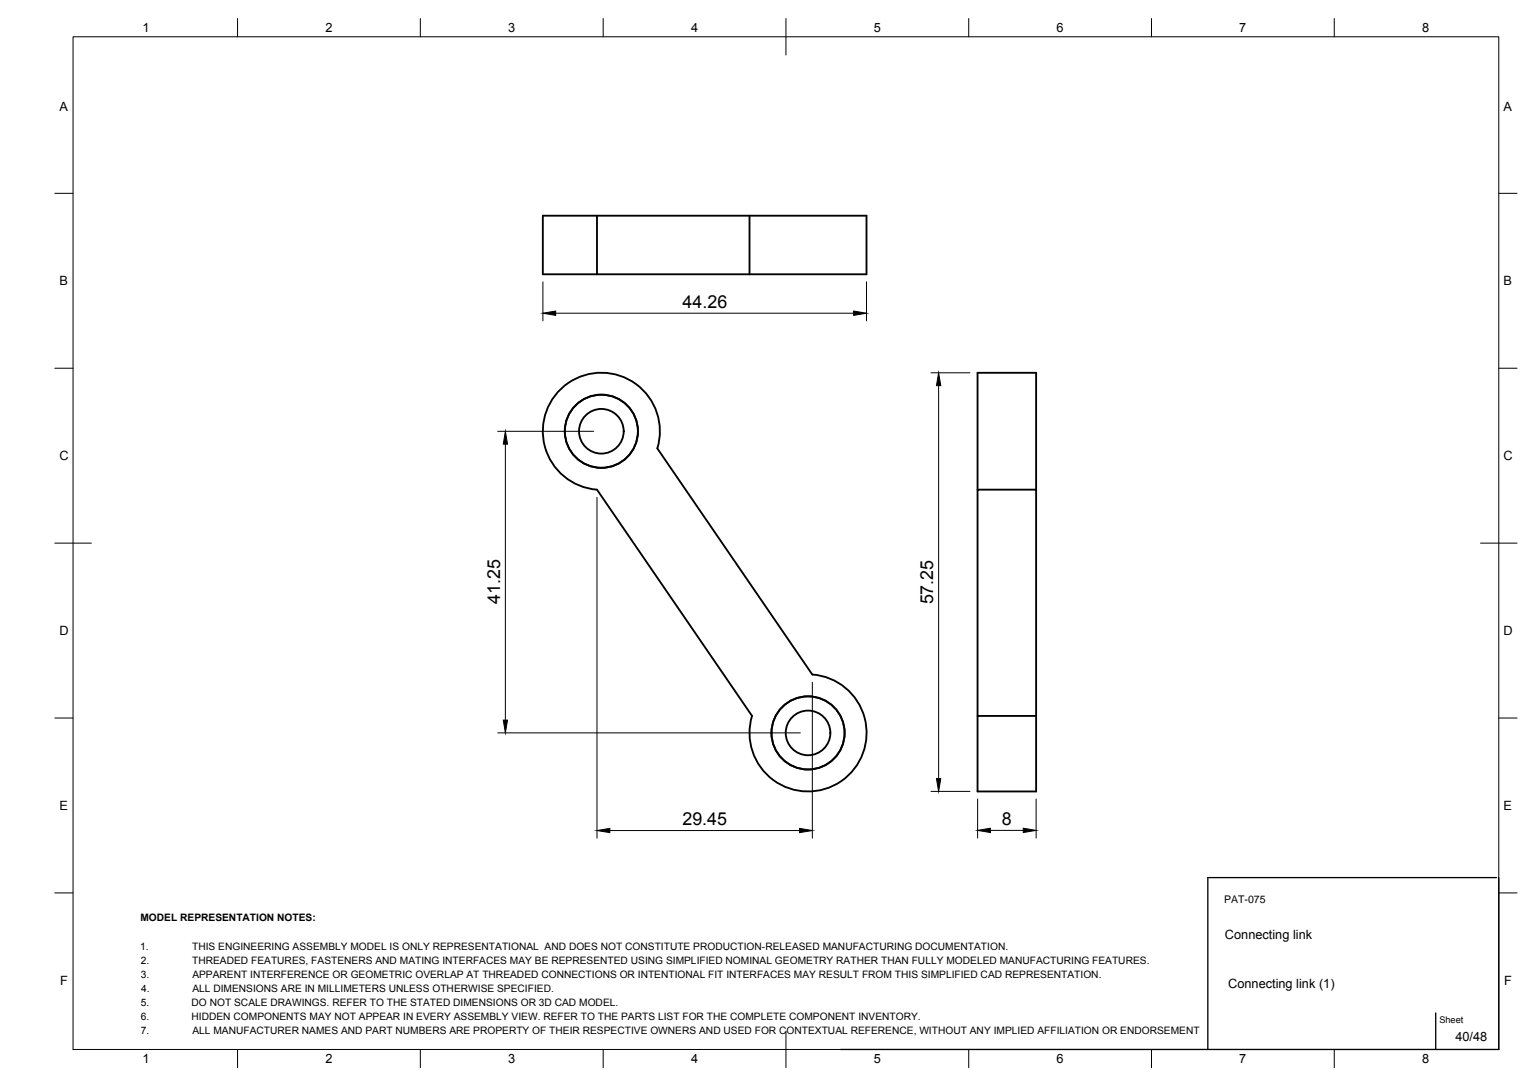
ISO-10303-21;
HEADER;
/* Generated by software containing ST-Developer
 * from STEP Tools, Inc. (www.steptools.com) 
 */

FILE_DESCRIPTION(
/* description */ ('Over-Centre Plunger Toggle Clamp on Slotted Fixture Frame'),
/* implementation_level */ '2;1');

FILE_NAME(
/* name */ 
'Connecting link.step',
/* time_stamp */ '2026-10-28T03:23:24-07:00',
/* author */ (''),
/* organization */ (''),
/* preprocessor_version */ 'ST-DEVELOPER v20.2',
/* originating_system */ 'Autodesk Translation Framework v15.17.0.0',
/* authorisation */ '');

FILE_SCHEMA (('AUTOMOTIVE_DESIGN { 1 0 10303 214 3 1 1 }'));
ENDSEC;

DATA;
#10=MECHANICAL_DESIGN_GEOMETRIC_PRESENTATION_REPRESENTATION('',(#556),#15212);
#464=SHAPE_REPRESENTATION_RELATIONSHIP('SRR','None',#15442,#506);
#506=ADVANCED_BREP_SHAPE_REPRESENTATION('',(#603),#15204);
#556=STYLED_ITEM('',(#15712),#603);
#603=MANIFOLD_SOLID_BREP('Body1',#8292);
#768=FACE_BOUND('',#2161,.T.);
#769=FACE_BOUND('',#2162,.T.);
#770=FACE_BOUND('',#2166,.T.);
#771=FACE_BOUND('',#2167,.T.);
#1046=PLANE('',#9644);
#1047=PLANE('',#9645);
#1048=PLANE('',#9647);
#1049=PLANE('',#9650);
#1513=FACE_OUTER_BOUND('',#2156,.T.);
#1514=FACE_OUTER_BOUND('',#2157,.T.);
#1515=FACE_OUTER_BOUND('',#2158,.T.);
#1516=FACE_OUTER_BOUND('',#2159,.T.);
#1517=FACE_OUTER_BOUND('',#2160,.T.);
#1518=FACE_OUTER_BOUND('',#2163,.T.);
#1519=FACE_OUTER_BOUND('',#2164,.T.);
#1520=FACE_OUTER_BOUND('',#2165,.T.);
#2156=EDGE_LOOP('',(#7377,#7378,#7379,#7380));
#2157=EDGE_LOOP('',(#7381,#7382,#7383,#7384));
#2158=EDGE_LOOP('',(#7385,#7386,#7387,#7388));
#2159=EDGE_LOOP('',(#7389,#7390,#7391,#7392));
#2160=EDGE_LOOP('',(#7393,#7394,#7395,#7396));
#2161=EDGE_LOOP('',(#7397));
#2162=EDGE_LOOP('',(#7398));
#2163=EDGE_LOOP('',(#7399,#7400,#7401,#7402));
#2164=EDGE_LOOP('',(#7403,#7404,#7405,#7406));
#2165=EDGE_LOOP('',(#7407,#7408,#7409,#7410));
#2166=EDGE_LOOP('',(#7411));
#2167=EDGE_LOOP('',(#7412));
#2784=LINE('',#14822,#3414);
#2785=LINE('',#14828,#3415);
#2786=LINE('',#14833,#3416);
#2787=LINE('',#14837,#3417);
#2788=LINE('',#14841,#3418);
#2789=LINE('',#14843,#3419);
#2790=LINE('',#14844,#3420);
#2791=LINE('',#14847,#3421);
#2792=LINE('',#14851,#3422);
#2793=LINE('',#14852,#3423);
#3414=VECTOR('',#12055,0.5);
#3415=VECTOR('',#12062,0.5);
#3416=VECTOR('',#12067,1.);
#3417=VECTOR('',#12070,1.);
#3418=VECTOR('',#12075,1.);
#3419=VECTOR('',#12076,1.);
#3420=VECTOR('',#12077,1.);
#3421=VECTOR('',#12080,1.);
#3422=VECTOR('',#12085,1.);
#3423=VECTOR('',#12086,1.);
#3818=CIRCLE('',#9636,0.5);
#3819=CIRCLE('',#9637,0.5);
#3820=CIRCLE('',#9639,0.5);
#3821=CIRCLE('',#9640,0.5);
#3822=CIRCLE('',#9642,0.8);
#3823=CIRCLE('',#9643,0.8);
#3824=CIRCLE('',#9646,0.8);
#3825=CIRCLE('',#9649,0.8);
#4466=VERTEX_POINT('',#14819);
#4467=VERTEX_POINT('',#14821);
#4468=VERTEX_POINT('',#14825);
#4469=VERTEX_POINT('',#14827);
#4470=VERTEX_POINT('',#14831);
#4471=VERTEX_POINT('',#14832);
#4472=VERTEX_POINT('',#14834);
#4473=VERTEX_POINT('',#14836);
#4474=VERTEX_POINT('',#14840);
#4475=VERTEX_POINT('',#14842);
#4476=VERTEX_POINT('',#14846);
#4477=VERTEX_POINT('',#14850);
#5449=EDGE_CURVE('',#4466,#4466,#3818,.T.);
#5450=EDGE_CURVE('',#4466,#4467,#2784,.T.);
#5451=EDGE_CURVE('',#4467,#4467,#3819,.T.);
#5452=EDGE_CURVE('',#4468,#4468,#3820,.T.);
#5453=EDGE_CURVE('',#4468,#4469,#2785,.T.);
#5454=EDGE_CURVE('',#4469,#4469,#3821,.T.);
#5455=EDGE_CURVE('',#4470,#4471,#2786,.T.);
#5456=EDGE_CURVE('',#4472,#4470,#3822,.T.);
#5457=EDGE_CURVE('',#4473,#4472,#2787,.T.);
#5458=EDGE_CURVE('',#4473,#4471,#3823,.T.);
#5459=EDGE_CURVE('',#4471,#4474,#2788,.T.);
#5460=EDGE_CURVE('',#4475,#4474,#2789,.T.);
#5461=EDGE_CURVE('',#4470,#4475,#2790,.T.);
#5462=EDGE_CURVE('',#4476,#4473,#2791,.T.);
#5463=EDGE_CURVE('',#4474,#4476,#3824,.T.);
#5464=EDGE_CURVE('',#4477,#4472,#2792,.T.);
#5465=EDGE_CURVE('',#4476,#4477,#2793,.T.);
#5466=EDGE_CURVE('',#4475,#4477,#3825,.T.);
#7377=ORIENTED_EDGE('',*,*,#5449,.F.);
#7378=ORIENTED_EDGE('',*,*,#5450,.T.);
#7379=ORIENTED_EDGE('',*,*,#5451,.F.);
#7380=ORIENTED_EDGE('',*,*,#5450,.F.);
#7381=ORIENTED_EDGE('',*,*,#5452,.F.);
#7382=ORIENTED_EDGE('',*,*,#5453,.T.);
#7383=ORIENTED_EDGE('',*,*,#5454,.F.);
#7384=ORIENTED_EDGE('',*,*,#5453,.F.);
#7385=ORIENTED_EDGE('',*,*,#5455,.F.);
#7386=ORIENTED_EDGE('',*,*,#5456,.F.);
#7387=ORIENTED_EDGE('',*,*,#5457,.F.);
#7388=ORIENTED_EDGE('',*,*,#5458,.T.);
#7389=ORIENTED_EDGE('',*,*,#5455,.T.);
#7390=ORIENTED_EDGE('',*,*,#5459,.T.);
#7391=ORIENTED_EDGE('',*,*,#5460,.F.);
#7392=ORIENTED_EDGE('',*,*,#5461,.F.);
#7393=ORIENTED_EDGE('',*,*,#5458,.F.);
#7394=ORIENTED_EDGE('',*,*,#5462,.F.);
#7395=ORIENTED_EDGE('',*,*,#5463,.F.);
#7396=ORIENTED_EDGE('',*,*,#5459,.F.);
#7397=ORIENTED_EDGE('',*,*,#5449,.T.);
#7398=ORIENTED_EDGE('',*,*,#5452,.T.);
#7399=ORIENTED_EDGE('',*,*,#5457,.T.);
#7400=ORIENTED_EDGE('',*,*,#5464,.F.);
#7401=ORIENTED_EDGE('',*,*,#5465,.F.);
#7402=ORIENTED_EDGE('',*,*,#5462,.T.);
#7403=ORIENTED_EDGE('',*,*,#5460,.T.);
#7404=ORIENTED_EDGE('',*,*,#5463,.T.);
#7405=ORIENTED_EDGE('',*,*,#5465,.T.);
#7406=ORIENTED_EDGE('',*,*,#5466,.F.);
#7407=ORIENTED_EDGE('',*,*,#5461,.T.);
#7408=ORIENTED_EDGE('',*,*,#5466,.T.);
#7409=ORIENTED_EDGE('',*,*,#5464,.T.);
#7410=ORIENTED_EDGE('',*,*,#5456,.T.);
#7411=ORIENTED_EDGE('',*,*,#5451,.T.);
#7412=ORIENTED_EDGE('',*,*,#5454,.T.);
#7742=CYLINDRICAL_SURFACE('',#9635,0.5);
#7743=CYLINDRICAL_SURFACE('',#9638,0.5);
#7744=CYLINDRICAL_SURFACE('',#9641,0.8);
#7745=CYLINDRICAL_SURFACE('',#9648,0.8);
#8185=ADVANCED_FACE('',(#1513),#7742,.F.);
#8186=ADVANCED_FACE('',(#1514),#7743,.F.);
#8187=ADVANCED_FACE('',(#1515),#7744,.T.);
#8188=ADVANCED_FACE('',(#1516),#1046,.T.);
#8189=ADVANCED_FACE('',(#1517,#768,#769),#1047,.F.);
#8190=ADVANCED_FACE('',(#1518),#1048,.T.);
#8191=ADVANCED_FACE('',(#1519),#7745,.T.);
#8192=ADVANCED_FACE('',(#1520,#770,#771),#1049,.T.);
#8292=CLOSED_SHELL('',(#8185,#8186,#8187,#8188,#8189,#8190,#8191,#8192));
#9634=AXIS2_PLACEMENT_3D('',#14817,#12049,#12050);
#9635=AXIS2_PLACEMENT_3D('',#14818,#12051,#12052);
#9636=AXIS2_PLACEMENT_3D('',#14820,#12053,#12054);
#9637=AXIS2_PLACEMENT_3D('',#14823,#12056,#12057);
#9638=AXIS2_PLACEMENT_3D('',#14824,#12058,#12059);
#9639=AXIS2_PLACEMENT_3D('',#14826,#12060,#12061);
#9640=AXIS2_PLACEMENT_3D('',#14829,#12063,#12064);
#9641=AXIS2_PLACEMENT_3D('',#14830,#12065,#12066);
#9642=AXIS2_PLACEMENT_3D('',#14835,#12068,#12069);
#9643=AXIS2_PLACEMENT_3D('',#14838,#12071,#12072);
#9644=AXIS2_PLACEMENT_3D('',#14839,#12073,#12074);
#9645=AXIS2_PLACEMENT_3D('',#14845,#12078,#12079);
#9646=AXIS2_PLACEMENT_3D('',#14848,#12081,#12082);
#9647=AXIS2_PLACEMENT_3D('',#14849,#12083,#12084);
#9648=AXIS2_PLACEMENT_3D('',#14853,#12087,#12088);
#9649=AXIS2_PLACEMENT_3D('',#14854,#12089,#12090);
#9650=AXIS2_PLACEMENT_3D('',#14855,#12091,#12092);
#12049=DIRECTION('axis',(0.,0.,1.));
#12050=DIRECTION('refdir',(1.,0.,0.));
#12051=DIRECTION('center_axis',(0.,1.,0.));
#12052=DIRECTION('ref_axis',(1.,0.,0.));
#12053=DIRECTION('center_axis',(0.,1.,0.));
#12054=DIRECTION('ref_axis',(1.,0.,0.));
#12055=DIRECTION('',(0.,1.,0.));
#12056=DIRECTION('center_axis',(0.,-1.,0.));
#12057=DIRECTION('ref_axis',(1.,0.,0.));
#12058=DIRECTION('center_axis',(0.,1.,0.));
#12059=DIRECTION('ref_axis',(1.,0.,0.));
#12060=DIRECTION('center_axis',(0.,1.,0.));
#12061=DIRECTION('ref_axis',(1.,0.,0.));
#12062=DIRECTION('',(0.,1.,0.));
#12063=DIRECTION('center_axis',(0.,-1.,0.));
#12064=DIRECTION('ref_axis',(1.,0.,0.));
#12065=DIRECTION('center_axis',(0.,1.,0.));
#12066=DIRECTION('ref_axis',(0.565264218607056,0.,-0.824909912149536));
#12067=DIRECTION('',(0.,-1.,0.));
#12068=DIRECTION('center_axis',(0.,1.,0.));
#12069=DIRECTION('ref_axis',(1.,0.,0.));
#12070=DIRECTION('',(0.,1.,0.));
#12071=DIRECTION('center_axis',(0.,1.,0.));
#12072=DIRECTION('ref_axis',(1.,0.,0.));
#12073=DIRECTION('center_axis',(-0.824909912149536,0.,-0.565264218607055));
#12074=DIRECTION('ref_axis',(-0.565264218607055,0.,0.824909912149537));
#12075=DIRECTION('',(-0.565264218607055,0.,0.824909912149537));
#12076=DIRECTION('',(0.,-1.,0.));
#12077=DIRECTION('',(-0.565264218607055,0.,0.824909912149537));
#12078=DIRECTION('center_axis',(0.,1.,0.));
#12079=DIRECTION('ref_axis',(1.,0.,0.));
#12080=DIRECTION('',(0.565264218607055,0.,-0.824909912149537));
#12081=DIRECTION('center_axis',(0.,1.,0.));
#12082=DIRECTION('ref_axis',(1.,0.,0.));
#12083=DIRECTION('center_axis',(0.824909912149536,0.,0.565264218607055));
#12084=DIRECTION('ref_axis',(0.565264218607055,0.,-0.824909912149537));
#12085=DIRECTION('',(0.565264218607055,0.,-0.824909912149537));
#12086=DIRECTION('',(0.,1.,0.));
#12087=DIRECTION('center_axis',(0.,1.,0.));
#12088=DIRECTION('ref_axis',(-0.565264218607055,0.,0.824909912149536));
#12089=DIRECTION('center_axis',(0.,1.,0.));
#12090=DIRECTION('ref_axis',(1.,0.,0.));
#12091=DIRECTION('center_axis',(0.,1.,0.));
#12092=DIRECTION('ref_axis',(1.,0.,0.));
#14817=CARTESIAN_POINT('',(0.,0.,0.));
#14818=CARTESIAN_POINT('Origin',(-2.82632109303527,-5.6,8.79263101785268));
#14819=CARTESIAN_POINT('',(-3.32632109303527,-5.5,8.79263101785268));
#14820=CARTESIAN_POINT('Origin',(-2.82632109303527,-5.5,8.79263101785268));
#14821=CARTESIAN_POINT('',(-3.32632109303527,-4.7,8.79263101785268));
#14822=CARTESIAN_POINT('',(-3.32632109303527,-5.6,8.79263101785268));
#14823=CARTESIAN_POINT('Origin',(-2.82632109303527,-4.7,8.79263101785268));
#14824=CARTESIAN_POINT('Origin',(0.,-5.6,4.668081457105));
#14825=CARTESIAN_POINT('',(-0.5,-5.5,4.668081457105));
#14826=CARTESIAN_POINT('Origin',(0.,-5.5,4.668081457105));
#14827=CARTESIAN_POINT('',(-0.5,-4.7,4.668081457105));
#14828=CARTESIAN_POINT('',(-0.5,-5.6,4.668081457105));
#14829=CARTESIAN_POINT('Origin',(0.,-4.7,4.668081457105));
#14830=CARTESIAN_POINT('Origin',(0.,-5.5,4.668081457105));
#14831=CARTESIAN_POINT('',(-0.765462347451497,-4.7,4.90060542282476));
#14832=CARTESIAN_POINT('',(-0.765462347451497,-5.5,4.90060542282476));
#14833=CARTESIAN_POINT('',(-0.765462347451497,-5.5,4.90060542282476));
#14834=CARTESIAN_POINT('',(0.059447564698039,-4.7,5.46586964143181));
#14835=CARTESIAN_POINT('Origin',(0.,-4.7,4.668081457105));
#14836=CARTESIAN_POINT('',(0.059447564698039,-5.5,5.46586964143181));
#14837=CARTESIAN_POINT('',(0.059447564698039,-5.5,5.46586964143181));
#14838=CARTESIAN_POINT('Origin',(0.,-5.5,4.668081457105));
#14839=CARTESIAN_POINT('Origin',(-0.412454956074768,-5.5,4.38544934780147));
#14840=CARTESIAN_POINT('',(-2.88576865773331,-5.5,7.99484283352587));
#14841=CARTESIAN_POINT('',(-0.412454956074768,-5.5,4.38544934780147));
#14842=CARTESIAN_POINT('',(-2.88576865773331,-4.7,7.99484283352587));
#14843=CARTESIAN_POINT('',(-2.88576865773331,-5.5,7.99484283352587));
#14844=CARTESIAN_POINT('',(-0.412454956074768,-4.7,4.38544934780147));
#14845=CARTESIAN_POINT('Origin',(-2.82632109303527,-5.5,8.79263101785268));
#14846=CARTESIAN_POINT('',(-2.06085874558378,-5.5,8.56010705213293));
#14847=CARTESIAN_POINT('',(-2.4138661369605,-5.5,9.07526312715621));
#14848=CARTESIAN_POINT('Origin',(-2.82632109303527,-5.5,8.79263101785268));
#14849=CARTESIAN_POINT('Origin',(-2.4138661369605,-5.5,9.07526312715621));
#14850=CARTESIAN_POINT('',(-2.06085874558378,-4.7,8.56010705213293));
#14851=CARTESIAN_POINT('',(-2.4138661369605,-4.7,9.07526312715621));
#14852=CARTESIAN_POINT('',(-2.06085874558378,-5.5,8.56010705213293));
#14853=CARTESIAN_POINT('Origin',(-2.82632109303527,-5.5,8.79263101785268));
#14854=CARTESIAN_POINT('Origin',(-2.82632109303527,-4.7,8.79263101785268));
#14855=CARTESIAN_POINT('Origin',(-2.82632109303527,-4.7,8.79263101785268));
#15154=UNCERTAINTY_MEASURE_WITH_UNIT(LENGTH_MEASURE(0.001),#15213,
'DISTANCE_ACCURACY_VALUE',
'Maximum model space distance between geometric entities at asserted c
onnectivities');
#15162=UNCERTAINTY_MEASURE_WITH_UNIT(LENGTH_MEASURE(0.001),#15213,
'DISTANCE_ACCURACY_VALUE',
'Maximum model space distance between geometric entities at asserted c
onnectivities');
#15204=(
GEOMETRIC_REPRESENTATION_CONTEXT(3)
GLOBAL_UNCERTAINTY_ASSIGNED_CONTEXT((#15154))
GLOBAL_UNIT_ASSIGNED_CONTEXT((#15213,#15215,#15216))
REPRESENTATION_CONTEXT('','3D')
);
#15212=(
GEOMETRIC_REPRESENTATION_CONTEXT(3)
GLOBAL_UNCERTAINTY_ASSIGNED_CONTEXT((#15162))
GLOBAL_UNIT_ASSIGNED_CONTEXT((#15213,#15215,#15216))
REPRESENTATION_CONTEXT('','3D')
);
#15213=(
LENGTH_UNIT()
NAMED_UNIT(*)
SI_UNIT(.CENTI.,.METRE.)
);
#15215=(
NAMED_UNIT(*)
PLANE_ANGLE_UNIT()
SI_UNIT($,.RADIAN.)
);
#15216=(
NAMED_UNIT(*)
SI_UNIT($,.STERADIAN.)
SOLID_ANGLE_UNIT()
);
#15258=SHAPE_DEFINITION_REPRESENTATION(#15382,#15442);
#15382=PRODUCT_DEFINITION_SHAPE('',$,#15492);
#15442=SHAPE_REPRESENTATION('',(#9634),#15204);
#15450=PRODUCT_DEFINITION_CONTEXT('part definition',#15599,'design');
#15492=PRODUCT_DEFINITION('Connecting link','Connecting link',#15541,
#15450);
#15541=PRODUCT_DEFINITION_FORMATION('',$,#15642);
#15599=APPLICATION_CONTEXT(
'Core Data for Automotive Mechanical Design Process');
#15600=PRODUCT_CONTEXT('part definition',#15599,'mechanical');
#15642=PRODUCT('Connecting link','Connecting link','Connecting link',
(#15600));
#15706=COLOUR_RGB('Sky Blue',0.24,0.69,0.87);
#15707=FILL_AREA_STYLE_COLOUR('',#15706);
#15708=FILL_AREA_STYLE('',(#15707));
#15709=SURFACE_STYLE_FILL_AREA(#15708);
#15710=SURFACE_SIDE_STYLE('',(#15709));
#15711=SURFACE_STYLE_USAGE(.BOTH.,#15710);
#15712=PRESENTATION_STYLE_ASSIGNMENT((#15711));
ENDSEC;
END-ISO-10303-21;
